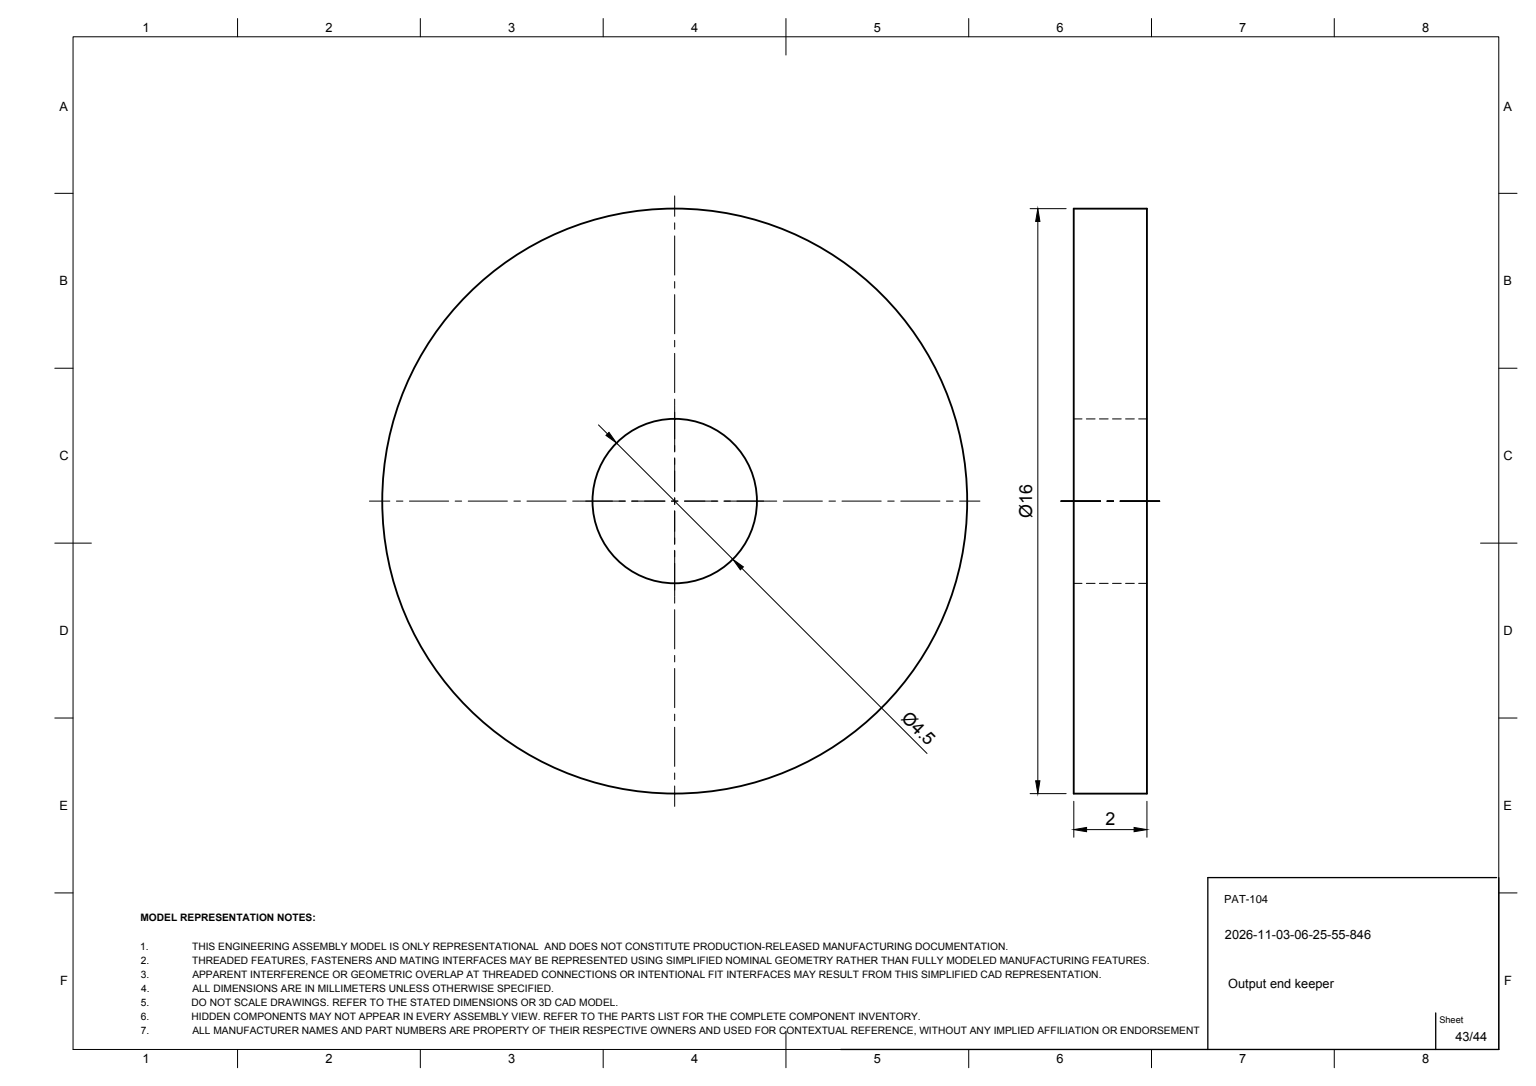
ISO-10303-21;
HEADER;
/* Generated by software containing ST-Developer
 * from STEP Tools, Inc. (www.steptools.com) 
 */

FILE_DESCRIPTION(
/* description */ ('Timing belt drive module 2 mm Pitch Timing 20T-40T'),

/* implementation_level */ '2;1');

FILE_NAME(
/* name */ 'Output end keeper.step',
/* time_stamp */ '2026-10-28T03:25:12-07:00',
/* author */ (''),
/* organization */ (''),
/* preprocessor_version */ 'ST-DEVELOPER v20.2',
/* originating_system */ 'Autodesk Translation Framework v15.17.0.0',
/* authorisation */ '');

FILE_SCHEMA (('AUTOMOTIVE_DESIGN { 1 0 10303 214 3 1 1 }'));
ENDSEC;

DATA;
#10=MECHANICAL_DESIGN_GEOMETRIC_PRESENTATION_REPRESENTATION('',(#579),#17830);
#478=SHAPE_REPRESENTATION_RELATIONSHIP('SRR','None',#18052,#521);
#521=ADVANCED_BREP_SHAPE_REPRESENTATION('',(#635),#17827);
#579=STYLED_ITEM('',(#18331),#635);
#635=MANIFOLD_SOLID_BREP('Body1',#9038);
#759=FACE_BOUND('',#2015,.T.);
#760=FACE_BOUND('',#2017,.T.);
#944=PLANE('',#10456);
#945=PLANE('',#10457);
#1369=FACE_OUTER_BOUND('',#2012,.T.);
#1370=FACE_OUTER_BOUND('',#2013,.T.);
#1371=FACE_OUTER_BOUND('',#2014,.T.);
#1372=FACE_OUTER_BOUND('',#2016,.T.);
#2012=EDGE_LOOP('',(#7545,#7546,#7547,#7548));
#2013=EDGE_LOOP('',(#7549,#7550,#7551,#7552));
#2014=EDGE_LOOP('',(#7553));
#2015=EDGE_LOOP('',(#7554));
#2016=EDGE_LOOP('',(#7555));
#2017=EDGE_LOOP('',(#7556));
#2610=CIRCLE('',#10451,0.225);
#2611=CIRCLE('',#10452,0.225);
#2612=CIRCLE('',#10454,0.8);
#2613=CIRCLE('',#10455,0.8);
#3152=LINE('',#16746,#3630);
#3153=LINE('',#16752,#3631);
#3630=VECTOR('',#13043,0.225);
#3631=VECTOR('',#13050,0.8);
#4355=VERTEX_POINT('',#16743);
#4356=VERTEX_POINT('',#16745);
#4357=VERTEX_POINT('',#16749);
#4358=VERTEX_POINT('',#16751);
#5455=EDGE_CURVE('',#4355,#4355,#2610,.T.);
#5456=EDGE_CURVE('',#4355,#4356,#3152,.T.);
#5457=EDGE_CURVE('',#4356,#4356,#2611,.T.);
#5458=EDGE_CURVE('',#4357,#4357,#2612,.T.);
#5459=EDGE_CURVE('',#4357,#4358,#3153,.T.);
#5460=EDGE_CURVE('',#4358,#4358,#2613,.T.);
#7545=ORIENTED_EDGE('',*,*,#5455,.F.);
#7546=ORIENTED_EDGE('',*,*,#5456,.T.);
#7547=ORIENTED_EDGE('',*,*,#5457,.T.);
#7548=ORIENTED_EDGE('',*,*,#5456,.F.);
#7549=ORIENTED_EDGE('',*,*,#5458,.F.);
#7550=ORIENTED_EDGE('',*,*,#5459,.T.);
#7551=ORIENTED_EDGE('',*,*,#5460,.T.);
#7552=ORIENTED_EDGE('',*,*,#5459,.F.);
#7553=ORIENTED_EDGE('',*,*,#5458,.T.);
#7554=ORIENTED_EDGE('',*,*,#5455,.T.);
#7555=ORIENTED_EDGE('',*,*,#5460,.F.);
#7556=ORIENTED_EDGE('',*,*,#5457,.F.);
#8368=CYLINDRICAL_SURFACE('',#10450,0.225);
#8369=CYLINDRICAL_SURFACE('',#10453,0.8);
#8867=ADVANCED_FACE('',(#1369),#8368,.F.);
#8868=ADVANCED_FACE('',(#1370),#8369,.T.);
#8869=ADVANCED_FACE('',(#1371,#759),#944,.T.);
#8870=ADVANCED_FACE('',(#1372,#760),#945,.F.);
#9038=CLOSED_SHELL('',(#8867,#8868,#8869,#8870));
#10449=AXIS2_PLACEMENT_3D('',#16741,#13037,#13038);
#10450=AXIS2_PLACEMENT_3D('',#16742,#13039,#13040);
#10451=AXIS2_PLACEMENT_3D('',#16744,#13041,#13042);
#10452=AXIS2_PLACEMENT_3D('',#16747,#13044,#13045);
#10453=AXIS2_PLACEMENT_3D('',#16748,#13046,#13047);
#10454=AXIS2_PLACEMENT_3D('',#16750,#13048,#13049);
#10455=AXIS2_PLACEMENT_3D('',#16753,#13051,#13052);
#10456=AXIS2_PLACEMENT_3D('',#16754,#13053,#13054);
#10457=AXIS2_PLACEMENT_3D('',#16755,#13055,#13056);
#13037=DIRECTION('axis',(0.,0.,1.));
#13038=DIRECTION('refdir',(1.,0.,0.));
#13039=DIRECTION('center_axis',(0.,1.,0.));
#13040=DIRECTION('ref_axis',(1.,0.,0.));
#13041=DIRECTION('center_axis',(0.,-1.,0.));
#13042=DIRECTION('ref_axis',(1.,0.,0.));
#13043=DIRECTION('',(0.,-1.,0.));
#13044=DIRECTION('center_axis',(0.,-1.,0.));
#13045=DIRECTION('ref_axis',(1.,0.,0.));
#13046=DIRECTION('center_axis',(0.,1.,0.));
#13047=DIRECTION('ref_axis',(1.,0.,0.));
#13048=DIRECTION('center_axis',(0.,1.,0.));
#13049=DIRECTION('ref_axis',(1.,0.,0.));
#13050=DIRECTION('',(0.,-1.,0.));
#13051=DIRECTION('center_axis',(0.,1.,0.));
#13052=DIRECTION('ref_axis',(1.,0.,0.));
#13053=DIRECTION('center_axis',(0.,1.,0.));
#13054=DIRECTION('ref_axis',(1.,0.,0.));
#13055=DIRECTION('center_axis',(0.,1.,0.));
#13056=DIRECTION('ref_axis',(1.,0.,0.));
#16741=CARTESIAN_POINT('',(0.,0.,0.));
#16742=CARTESIAN_POINT('Origin',(6.97091003018116,-5.2,7.));
#16743=CARTESIAN_POINT('',(6.74591003018116,-5.,7.));
#16744=CARTESIAN_POINT('Origin',(6.97091003018116,-5.,7.));
#16745=CARTESIAN_POINT('',(6.74591003018116,-5.2,7.));
#16746=CARTESIAN_POINT('',(6.74591003018116,-5.2,7.));
#16747=CARTESIAN_POINT('Origin',(6.97091003018116,-5.2,7.));
#16748=CARTESIAN_POINT('Origin',(6.97091003018116,-5.2,7.));
#16749=CARTESIAN_POINT('',(6.17091003018116,-5.,7.));
#16750=CARTESIAN_POINT('Origin',(6.97091003018116,-5.,7.));
#16751=CARTESIAN_POINT('',(6.17091003018116,-5.2,7.));
#16752=CARTESIAN_POINT('',(6.17091003018116,-5.2,7.));
#16753=CARTESIAN_POINT('Origin',(6.97091003018116,-5.2,7.));
#16754=CARTESIAN_POINT('Origin',(6.97091003018116,-5.,7.));
#16755=CARTESIAN_POINT('Origin',(6.97091003018116,-5.2,7.));
#17777=UNCERTAINTY_MEASURE_WITH_UNIT(LENGTH_MEASURE(0.001),#17831,
'DISTANCE_ACCURACY_VALUE',
'Maximum model space distance between geometric entities at asserted c
onnectivities');
#17780=UNCERTAINTY_MEASURE_WITH_UNIT(LENGTH_MEASURE(0.001),#17831,
'DISTANCE_ACCURACY_VALUE',
'Maximum model space distance between geometric entities at asserted c
onnectivities');
#17827=(
GEOMETRIC_REPRESENTATION_CONTEXT(3)
GLOBAL_UNCERTAINTY_ASSIGNED_CONTEXT((#17777))
GLOBAL_UNIT_ASSIGNED_CONTEXT((#17831,#17833,#17834))
REPRESENTATION_CONTEXT('','3D')
);
#17830=(
GEOMETRIC_REPRESENTATION_CONTEXT(3)
GLOBAL_UNCERTAINTY_ASSIGNED_CONTEXT((#17780))
GLOBAL_UNIT_ASSIGNED_CONTEXT((#17831,#17833,#17834))
REPRESENTATION_CONTEXT('','3D')
);
#17831=(
LENGTH_UNIT()
NAMED_UNIT(*)
SI_UNIT(.CENTI.,.METRE.)
);
#17833=(
NAMED_UNIT(*)
PLANE_ANGLE_UNIT()
SI_UNIT($,.RADIAN.)
);
#17834=(
NAMED_UNIT(*)
SI_UNIT($,.STERADIAN.)
SOLID_ANGLE_UNIT()
);
#17881=SHAPE_DEFINITION_REPRESENTATION(#17940,#18052);
#17940=PRODUCT_DEFINITION_SHAPE('',$,#18102);
#18052=SHAPE_REPRESENTATION('',(#10449),#17827);
#18055=PRODUCT_DEFINITION_CONTEXT('part definition',#18204,'design');
#18102=PRODUCT_DEFINITION('Output end keeper','Output end keeper',#18151,
#18055);
#18151=PRODUCT_DEFINITION_FORMATION('',$,#18252);
#18204=APPLICATION_CONTEXT(
'Core Data for Automotive Mechanical Design Process');
#18205=PRODUCT_CONTEXT('part definition',#18204,'mechanical');
#18252=PRODUCT('Output end keeper','Output end keeper',
'Output end keeper',(#18205));
#18325=COLOUR_RGB('Off White',0.89,0.88,0.83);
#18326=FILL_AREA_STYLE_COLOUR('',#18325);
#18327=FILL_AREA_STYLE('',(#18326));
#18328=SURFACE_STYLE_FILL_AREA(#18327);
#18329=SURFACE_SIDE_STYLE('',(#18328));
#18330=SURFACE_STYLE_USAGE(.BOTH.,#18329);
#18331=PRESENTATION_STYLE_ASSIGNMENT((#18330));
ENDSEC;
END-ISO-10303-21;
